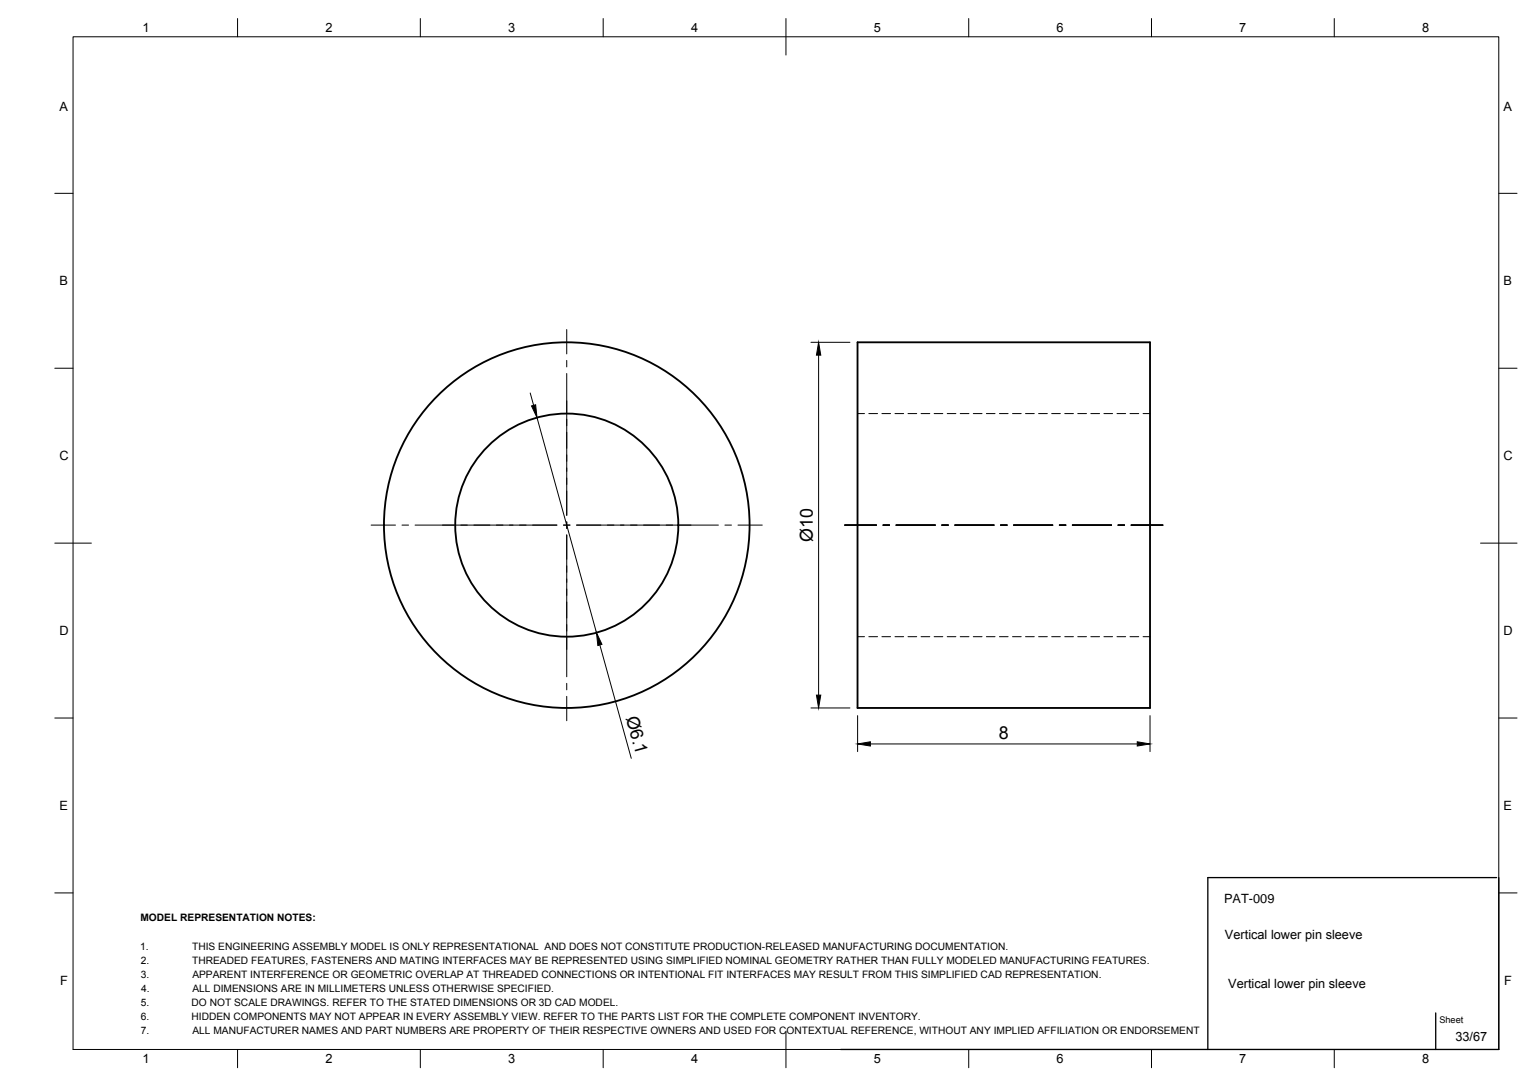
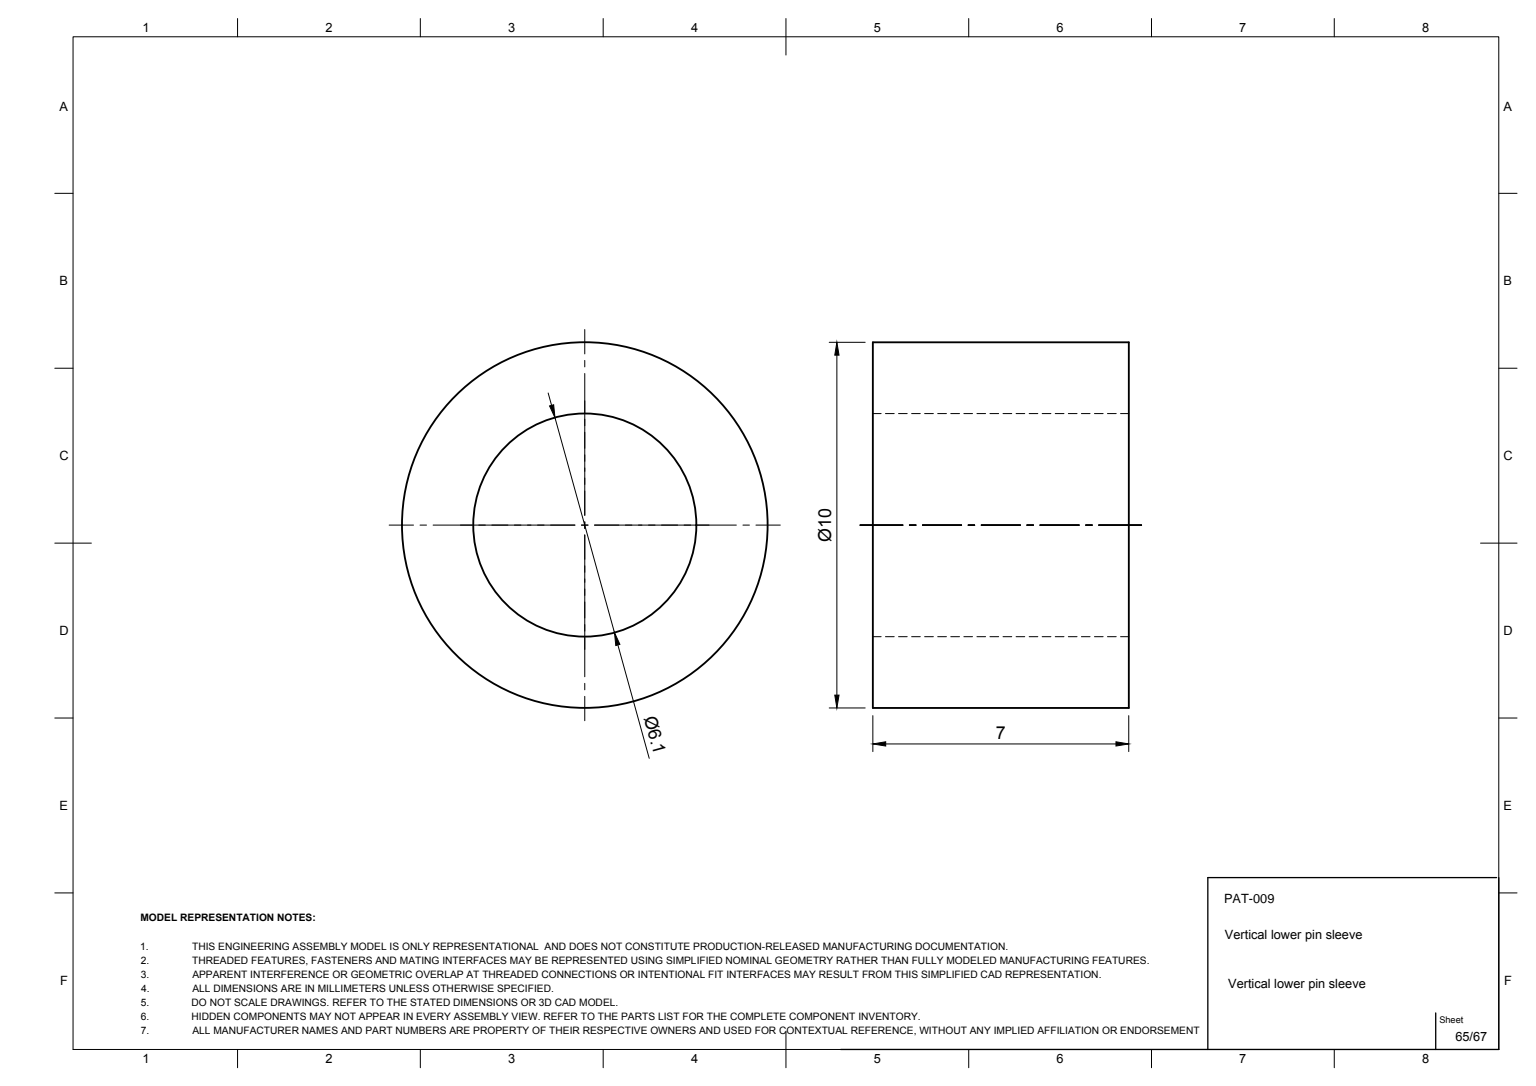
ISO-10303-21;
HEADER;
/* Generated by software containing ST-Developer
 * from STEP Tools, Inc. (www.steptools.com) 
 */

FILE_DESCRIPTION(
/* description */ ('Bell-crank linkage with push rods'),
/* implementation_level */ '2;1');

FILE_NAME(
/* name */ 'Vertical lower pin sleeve.step',
/* time_stamp */ '2026-10-28T03:25:15-07:00',
/* author */ (''),
/* organization */ (''),
/* preprocessor_version */ 'ST-DEVELOPER v20.2',
/* originating_system */ 'Autodesk Translation Framework v15.17.0.0',
/* authorisation */ '');

FILE_SCHEMA (('AUTOMOTIVE_DESIGN { 1 0 10303 214 3 1 1 }'));
ENDSEC;

DATA;
#10=MECHANICAL_DESIGN_GEOMETRIC_PRESENTATION_REPRESENTATION('',(#638),#16678);
#522=SHAPE_REPRESENTATION_RELATIONSHIP('SRR','None',#16940,#576);
#576=ADVANCED_BREP_SHAPE_REPRESENTATION('',(#699),#16645);
#638=STYLED_ITEM('',(#17291),#699);
#699=MANIFOLD_SOLID_BREP('Body1',#8829);
#850=FACE_BOUND('',#2194,.T.);
#851=FACE_BOUND('',#2196,.T.);
#1117=PLANE('',#10095);
#1118=PLANE('',#10096);
#1544=FACE_OUTER_BOUND('',#2191,.T.);
#1545=FACE_OUTER_BOUND('',#2192,.T.);
#1546=FACE_OUTER_BOUND('',#2193,.T.);
#1547=FACE_OUTER_BOUND('',#2195,.T.);
#2191=EDGE_LOOP('',(#7189,#7190,#7191,#7192));
#2192=EDGE_LOOP('',(#7193,#7194,#7195,#7196));
#2193=EDGE_LOOP('',(#7197));
#2194=EDGE_LOOP('',(#7198));
#2195=EDGE_LOOP('',(#7199));
#2196=EDGE_LOOP('',(#7200));
#2830=LINE('',#15473,#3379);
#2831=LINE('',#15479,#3380);
#3379=VECTOR('',#12202,0.305);
#3380=VECTOR('',#12209,0.5);
#3932=CIRCLE('',#10090,0.305);
#3933=CIRCLE('',#10091,0.305);
#3934=CIRCLE('',#10093,0.5);
#3935=CIRCLE('',#10094,0.5);
#4543=VERTEX_POINT('',#15470);
#4544=VERTEX_POINT('',#15472);
#4545=VERTEX_POINT('',#15476);
#4546=VERTEX_POINT('',#15478);
#5472=EDGE_CURVE('',#4543,#4543,#3932,.T.);
#5473=EDGE_CURVE('',#4543,#4544,#2830,.T.);
#5474=EDGE_CURVE('',#4544,#4544,#3933,.T.);
#5475=EDGE_CURVE('',#4545,#4545,#3934,.T.);
#5476=EDGE_CURVE('',#4545,#4546,#2831,.T.);
#5477=EDGE_CURVE('',#4546,#4546,#3935,.T.);
#7189=ORIENTED_EDGE('',*,*,#5472,.F.);
#7190=ORIENTED_EDGE('',*,*,#5473,.T.);
#7191=ORIENTED_EDGE('',*,*,#5474,.T.);
#7192=ORIENTED_EDGE('',*,*,#5473,.F.);
#7193=ORIENTED_EDGE('',*,*,#5475,.F.);
#7194=ORIENTED_EDGE('',*,*,#5476,.T.);
#7195=ORIENTED_EDGE('',*,*,#5477,.T.);
#7196=ORIENTED_EDGE('',*,*,#5476,.F.);
#7197=ORIENTED_EDGE('',*,*,#5475,.T.);
#7198=ORIENTED_EDGE('',*,*,#5472,.T.);
#7199=ORIENTED_EDGE('',*,*,#5477,.F.);
#7200=ORIENTED_EDGE('',*,*,#5474,.F.);
#8185=CYLINDRICAL_SURFACE('',#10089,0.305);
#8186=CYLINDRICAL_SURFACE('',#10092,0.5);
#8569=ADVANCED_FACE('',(#1544),#8185,.F.);
#8570=ADVANCED_FACE('',(#1545),#8186,.T.);
#8571=ADVANCED_FACE('',(#1546,#850),#1117,.T.);
#8572=ADVANCED_FACE('',(#1547,#851),#1118,.F.);
#8829=CLOSED_SHELL('',(#8569,#8570,#8571,#8572));
#10088=AXIS2_PLACEMENT_3D('',#15468,#12196,#12197);
#10089=AXIS2_PLACEMENT_3D('',#15469,#12198,#12199);
#10090=AXIS2_PLACEMENT_3D('',#15471,#12200,#12201);
#10091=AXIS2_PLACEMENT_3D('',#15474,#12203,#12204);
#10092=AXIS2_PLACEMENT_3D('',#15475,#12205,#12206);
#10093=AXIS2_PLACEMENT_3D('',#15477,#12207,#12208);
#10094=AXIS2_PLACEMENT_3D('',#15480,#12210,#12211);
#10095=AXIS2_PLACEMENT_3D('',#15481,#12212,#12213);
#10096=AXIS2_PLACEMENT_3D('',#15482,#12214,#12215);
#12196=DIRECTION('axis',(0.,0.,1.));
#12197=DIRECTION('refdir',(1.,0.,0.));
#12198=DIRECTION('center_axis',(0.,0.,1.));
#12199=DIRECTION('ref_axis',(1.,0.,0.));
#12200=DIRECTION('center_axis',(0.,0.,-1.));
#12201=DIRECTION('ref_axis',(1.,0.,0.));
#12202=DIRECTION('',(0.,0.,-1.));
#12203=DIRECTION('center_axis',(0.,0.,-1.));
#12204=DIRECTION('ref_axis',(1.,0.,0.));
#12205=DIRECTION('center_axis',(0.,0.,1.));
#12206=DIRECTION('ref_axis',(1.,0.,0.));
#12207=DIRECTION('center_axis',(0.,0.,1.));
#12208=DIRECTION('ref_axis',(1.,0.,0.));
#12209=DIRECTION('',(0.,0.,-1.));
#12210=DIRECTION('center_axis',(0.,0.,1.));
#12211=DIRECTION('ref_axis',(1.,0.,0.));
#12212=DIRECTION('center_axis',(0.,0.,1.));
#12213=DIRECTION('ref_axis',(1.,0.,0.));
#12214=DIRECTION('center_axis',(0.,0.,1.));
#12215=DIRECTION('ref_axis',(1.,0.,0.));
#15468=CARTESIAN_POINT('',(0.,0.,0.));
#15469=CARTESIAN_POINT('Origin',(4.,0.,6.));
#15470=CARTESIAN_POINT('',(3.695,-3.73517273739942E-17,6.8));
#15471=CARTESIAN_POINT('Origin',(4.,0.,6.8));
#15472=CARTESIAN_POINT('',(3.695,-3.73517273739942E-17,6.));
#15473=CARTESIAN_POINT('',(3.695,-3.73517273739942E-17,6.));
#15474=CARTESIAN_POINT('Origin',(4.,0.,6.));
#15475=CARTESIAN_POINT('Origin',(4.,0.,6.));
#15476=CARTESIAN_POINT('',(3.5,-6.12323399573677E-17,6.8));
#15477=CARTESIAN_POINT('Origin',(4.,0.,6.8));
#15478=CARTESIAN_POINT('',(3.5,-6.12323399573677E-17,6.));
#15479=CARTESIAN_POINT('',(3.5,-6.12323399573677E-17,6.));
#15480=CARTESIAN_POINT('Origin',(4.,0.,6.));
#15481=CARTESIAN_POINT('Origin',(4.,0.,6.8));
#15482=CARTESIAN_POINT('Origin',(4.,0.,6.));
#16581=UNCERTAINTY_MEASURE_WITH_UNIT(LENGTH_MEASURE(0.001),#16679,
'DISTANCE_ACCURACY_VALUE',
'Maximum model space distance between geometric entities at asserted c
onnectivities');
#16614=UNCERTAINTY_MEASURE_WITH_UNIT(LENGTH_MEASURE(0.001),#16679,
'DISTANCE_ACCURACY_VALUE',
'Maximum model space distance between geometric entities at asserted c
onnectivities');
#16645=(
GEOMETRIC_REPRESENTATION_CONTEXT(3)
GLOBAL_UNCERTAINTY_ASSIGNED_CONTEXT((#16581))
GLOBAL_UNIT_ASSIGNED_CONTEXT((#16679,#16681,#16682))
REPRESENTATION_CONTEXT('','3D')
);
#16678=(
GEOMETRIC_REPRESENTATION_CONTEXT(3)
GLOBAL_UNCERTAINTY_ASSIGNED_CONTEXT((#16614))
GLOBAL_UNIT_ASSIGNED_CONTEXT((#16679,#16681,#16682))
REPRESENTATION_CONTEXT('','3D')
);
#16679=(
LENGTH_UNIT()
NAMED_UNIT(*)
SI_UNIT(.CENTI.,.METRE.)
);
#16681=(
NAMED_UNIT(*)
PLANE_ANGLE_UNIT()
SI_UNIT($,.RADIAN.)
);
#16682=(
NAMED_UNIT(*)
SI_UNIT($,.STERADIAN.)
SOLID_ANGLE_UNIT()
);
#16713=SHAPE_DEFINITION_REPRESENTATION(#16781,#16940);
#16781=PRODUCT_DEFINITION_SHAPE('',$,#17004);
#16940=SHAPE_REPRESENTATION('',(#10088),#16645);
#16973=PRODUCT_DEFINITION_CONTEXT('part definition',#17164,'design');
#17004=PRODUCT_DEFINITION('Vertical lower pin sleeve',
'Vertical lower pin sleeve',#17067,#16973);
#17067=PRODUCT_DEFINITION_FORMATION('',$,#17196);
#17164=APPLICATION_CONTEXT(
'Core Data for Automotive Mechanical Design Process');
#17165=PRODUCT_CONTEXT('part definition',#17164,'mechanical');
#17196=PRODUCT('Vertical lower pin sleeve','Vertical lower pin sleeve',
'Vertical lower pin sleeve',(#17165));
#17285=COLOUR_RGB('Grey',0.48,0.52,0.57);
#17286=FILL_AREA_STYLE_COLOUR('',#17285);
#17287=FILL_AREA_STYLE('',(#17286));
#17288=SURFACE_STYLE_FILL_AREA(#17287);
#17289=SURFACE_SIDE_STYLE('',(#17288));
#17290=SURFACE_STYLE_USAGE(.BOTH.,#17289);
#17291=PRESENTATION_STYLE_ASSIGNMENT((#17290));
ENDSEC;
END-ISO-10303-21;
